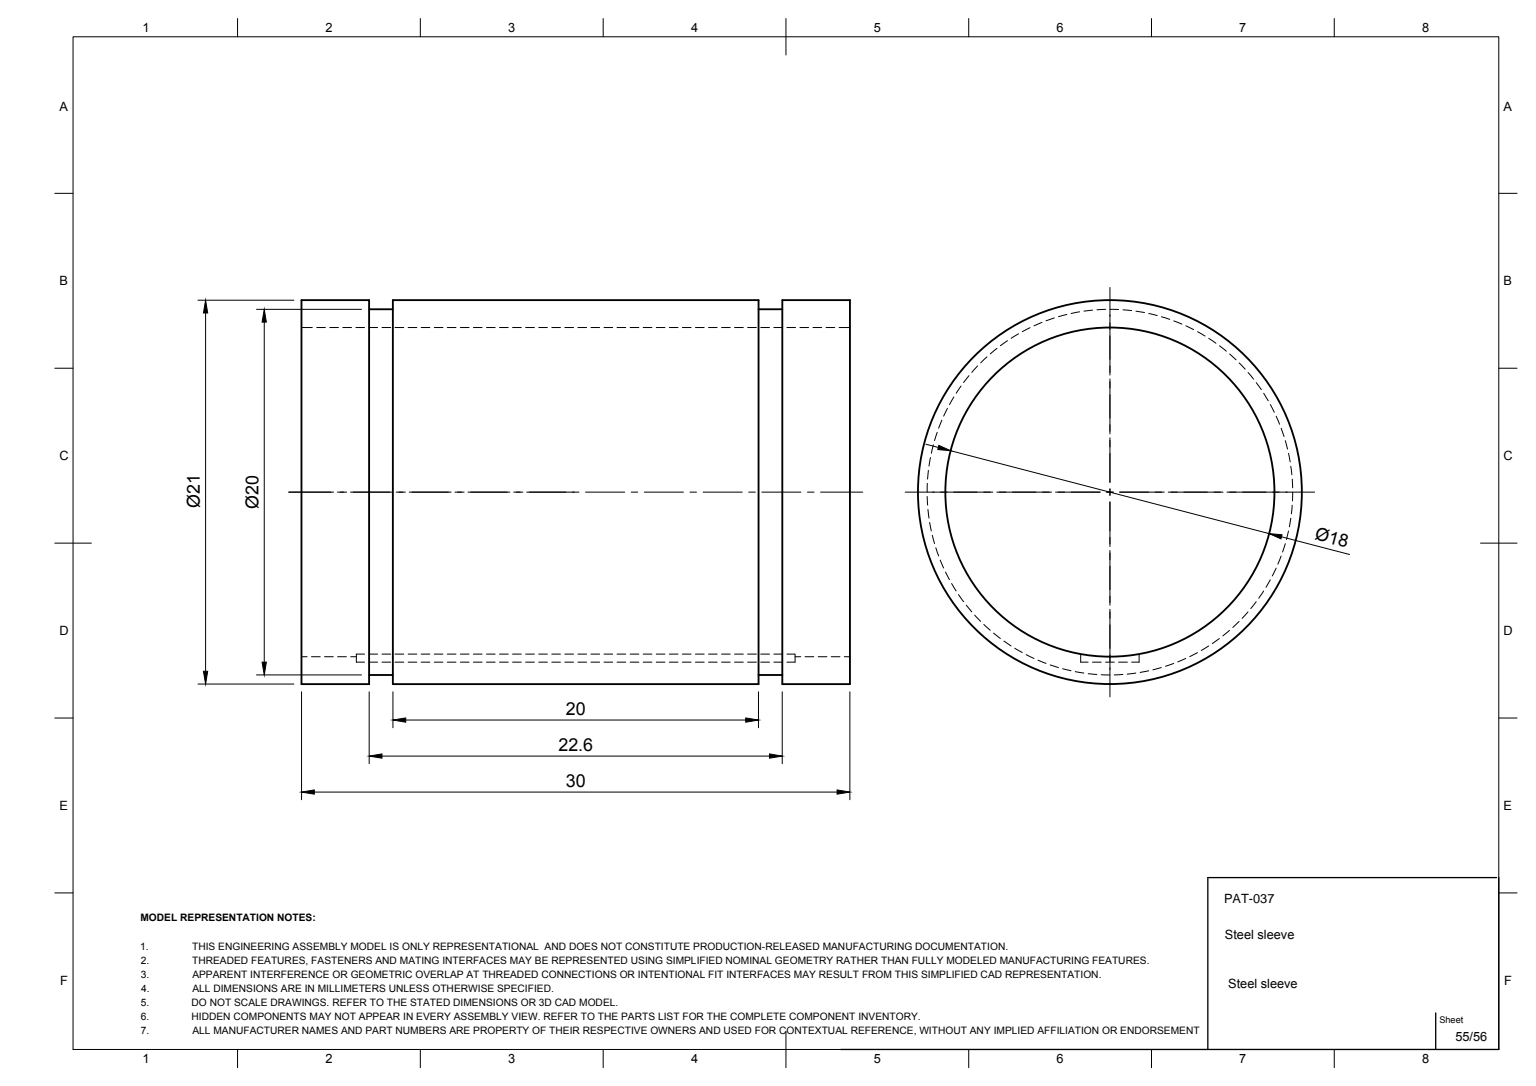
ISO-10303-21;
HEADER;
/* Generated by software containing ST-Developer
 * from STEP Tools, Inc. (www.steptools.com) 
 */

FILE_DESCRIPTION(
/* description */ ('Flywheel Crank-Slider'),
/* implementation_level */ '2;1');

FILE_NAME(
/* name */ 'Steel sleeve.step',
/* time_stamp */ '2026-10-28T03:23:13-07:00',
/* author */ (''),
/* organization */ (''),
/* preprocessor_version */ 'ST-DEVELOPER v20.2',
/* originating_system */ 'Autodesk Translation Framework v15.17.0.0',
/* authorisation */ '');

FILE_SCHEMA (('AUTOMOTIVE_DESIGN { 1 0 10303 214 3 1 1 }'));
ENDSEC;

DATA;
#10=MECHANICAL_DESIGN_GEOMETRIC_PRESENTATION_REPRESENTATION('',(#726),#17322);
#613=SHAPE_REPRESENTATION_RELATIONSHIP('SRR','None',#17615,#665);
#665=ADVANCED_BREP_SHAPE_REPRESENTATION('',(#783),#17319);
#726=STYLED_ITEM('',(#17945),#783);
#783=MANIFOLD_SOLID_BREP('Body1',#9108);
#999=FACE_BOUND('',#2569,.T.);
#1000=FACE_BOUND('',#2572,.T.);
#1001=FACE_BOUND('',#2575,.T.);
#1002=FACE_BOUND('',#2578,.T.);
#1003=FACE_BOUND('',#2581,.T.);
#1004=FACE_BOUND('',#2584,.T.);
#1005=FACE_BOUND('',#2586,.T.);
#1292=PLANE('',#10661);
#1293=PLANE('',#10663);
#1294=PLANE('',#10664);
#1295=PLANE('',#10666);
#1296=PLANE('',#10667);
#1297=PLANE('',#10668);
#1298=PLANE('',#10673);
#1299=PLANE('',#10677);
#1300=PLANE('',#10681);
#1301=PLANE('',#10685);
#1302=PLANE('',#10689);
#1814=FACE_OUTER_BOUND('',#2563,.T.);
#1815=FACE_OUTER_BOUND('',#2564,.T.);
#1816=FACE_OUTER_BOUND('',#2565,.T.);
#1817=FACE_OUTER_BOUND('',#2566,.T.);
#1818=FACE_OUTER_BOUND('',#2567,.T.);
#1819=FACE_OUTER_BOUND('',#2568,.T.);
#1820=FACE_OUTER_BOUND('',#2570,.T.);
#1821=FACE_OUTER_BOUND('',#2571,.T.);
#1822=FACE_OUTER_BOUND('',#2573,.T.);
#1823=FACE_OUTER_BOUND('',#2574,.T.);
#1824=FACE_OUTER_BOUND('',#2576,.T.);
#1825=FACE_OUTER_BOUND('',#2577,.T.);
#1826=FACE_OUTER_BOUND('',#2579,.T.);
#1827=FACE_OUTER_BOUND('',#2580,.T.);
#1828=FACE_OUTER_BOUND('',#2582,.T.);
#1829=FACE_OUTER_BOUND('',#2583,.T.);
#1830=FACE_OUTER_BOUND('',#2585,.T.);
#2563=EDGE_LOOP('',(#8174,#8175,#8176,#8177));
#2564=EDGE_LOOP('',(#8178,#8179,#8180,#8181));
#2565=EDGE_LOOP('',(#8182,#8183,#8184,#8185));
#2566=EDGE_LOOP('',(#8186,#8187,#8188,#8189));
#2567=EDGE_LOOP('',(#8190,#8191,#8192,#8193));
#2568=EDGE_LOOP('',(#8194));
#2569=EDGE_LOOP('',(#8195));
#2570=EDGE_LOOP('',(#8196,#8197,#8198,#8199));
#2571=EDGE_LOOP('',(#8200));
#2572=EDGE_LOOP('',(#8201));
#2573=EDGE_LOOP('',(#8202,#8203,#8204,#8205));
#2574=EDGE_LOOP('',(#8206));
#2575=EDGE_LOOP('',(#8207));
#2576=EDGE_LOOP('',(#8208,#8209,#8210,#8211));
#2577=EDGE_LOOP('',(#8212));
#2578=EDGE_LOOP('',(#8213));
#2579=EDGE_LOOP('',(#8214,#8215,#8216,#8217));
#2580=EDGE_LOOP('',(#8218));
#2581=EDGE_LOOP('',(#8219));
#2582=EDGE_LOOP('',(#8220,#8221,#8222,#8223));
#2583=EDGE_LOOP('',(#8224));
#2584=EDGE_LOOP('',(#8225));
#2585=EDGE_LOOP('',(#8226,#8227,#8228,#8229));
#2586=EDGE_LOOP('',(#8230,#8231,#8232,#8233));
#3178=LINE('',#16937,#3789);
#3179=LINE('',#16939,#3790);
#3180=LINE('',#16940,#3791);
#3181=LINE('',#16943,#3792);
#3182=LINE('',#16945,#3793);
#3183=LINE('',#16946,#3794);
#3184=LINE('',#16951,#3795);
#3185=LINE('',#16952,#3796);
#3186=LINE('',#16954,#3797);
#3187=LINE('',#16955,#3798);
#3188=LINE('',#16965,#3799);
#3189=LINE('',#16972,#3800);
#3190=LINE('',#16979,#3801);
#3191=LINE('',#16986,#3802);
#3192=LINE('',#16993,#3803);
#3193=LINE('',#16998,#3804);
#3789=VECTOR('',#13348,1.);
#3790=VECTOR('',#13349,1.);
#3791=VECTOR('',#13350,1.);
#3792=VECTOR('',#13353,1.);
#3793=VECTOR('',#13354,1.);
#3794=VECTOR('',#13355,1.);
#3795=VECTOR('',#13360,1.);
#3796=VECTOR('',#13361,1.);
#3797=VECTOR('',#13364,1.);
#3798=VECTOR('',#13365,1.);
#3799=VECTOR('',#13378,1.05);
#3800=VECTOR('',#13387,1.);
#3801=VECTOR('',#13396,1.05);
#3802=VECTOR('',#13405,1.);
#3803=VECTOR('',#13414,1.05);
#3804=VECTOR('',#13421,0.9);
#4248=CIRCLE('',#10662,0.9);
#4249=CIRCLE('',#10665,0.9);
#4250=CIRCLE('',#10669,1.05);
#4251=CIRCLE('',#10670,0.9);
#4252=CIRCLE('',#10672,1.05);
#4253=CIRCLE('',#10674,1.);
#4254=CIRCLE('',#10676,1.);
#4255=CIRCLE('',#10678,1.05);
#4256=CIRCLE('',#10680,1.05);
#4257=CIRCLE('',#10682,1.);
#4258=CIRCLE('',#10684,1.);
#4259=CIRCLE('',#10686,1.05);
#4260=CIRCLE('',#10688,1.05);
#4261=CIRCLE('',#10690,0.9);
#4967=VERTEX_POINT('',#16933);
#4968=VERTEX_POINT('',#16934);
#4969=VERTEX_POINT('',#16936);
#4970=VERTEX_POINT('',#16938);
#4971=VERTEX_POINT('',#16942);
#4972=VERTEX_POINT('',#16944);
#4973=VERTEX_POINT('',#16948);
#4974=VERTEX_POINT('',#16950);
#4975=VERTEX_POINT('',#16958);
#4976=VERTEX_POINT('',#16960);
#4977=VERTEX_POINT('',#16963);
#4978=VERTEX_POINT('',#16967);
#4979=VERTEX_POINT('',#16970);
#4980=VERTEX_POINT('',#16974);
#4981=VERTEX_POINT('',#16977);
#4982=VERTEX_POINT('',#16981);
#4983=VERTEX_POINT('',#16984);
#4984=VERTEX_POINT('',#16988);
#4985=VERTEX_POINT('',#16991);
#4986=VERTEX_POINT('',#16995);
#6044=EDGE_CURVE('',#4967,#4968,#4248,.T.);
#6045=EDGE_CURVE('',#4969,#4967,#3178,.T.);
#6046=EDGE_CURVE('',#4970,#4969,#3179,.T.);
#6047=EDGE_CURVE('',#4968,#4970,#3180,.T.);
#6048=EDGE_CURVE('',#4968,#4971,#3181,.T.);
#6049=EDGE_CURVE('',#4972,#4970,#3182,.T.);
#6050=EDGE_CURVE('',#4972,#4971,#3183,.T.);
#6051=EDGE_CURVE('',#4971,#4973,#4249,.T.);
#6052=EDGE_CURVE('',#4974,#4972,#3184,.T.);
#6053=EDGE_CURVE('',#4973,#4974,#3185,.T.);
#6054=EDGE_CURVE('',#4973,#4967,#3186,.T.);
#6055=EDGE_CURVE('',#4974,#4969,#3187,.T.);
#6056=EDGE_CURVE('',#4975,#4975,#4250,.T.);
#6057=EDGE_CURVE('',#4976,#4976,#4251,.T.);
#6058=EDGE_CURVE('',#4977,#4977,#4252,.T.);
#6059=EDGE_CURVE('',#4977,#4975,#3188,.T.);
#6060=EDGE_CURVE('',#4978,#4978,#4253,.T.);
#6061=EDGE_CURVE('',#4979,#4979,#4254,.T.);
#6062=EDGE_CURVE('',#4979,#4978,#3189,.T.);
#6063=EDGE_CURVE('',#4980,#4980,#4255,.T.);
#6064=EDGE_CURVE('',#4981,#4981,#4256,.T.);
#6065=EDGE_CURVE('',#4981,#4980,#3190,.T.);
#6066=EDGE_CURVE('',#4982,#4982,#4257,.T.);
#6067=EDGE_CURVE('',#4983,#4983,#4258,.T.);
#6068=EDGE_CURVE('',#4983,#4982,#3191,.T.);
#6069=EDGE_CURVE('',#4984,#4984,#4259,.T.);
#6070=EDGE_CURVE('',#4985,#4985,#4260,.T.);
#6071=EDGE_CURVE('',#4985,#4984,#3192,.T.);
#6072=EDGE_CURVE('',#4986,#4986,#4261,.T.);
#6073=EDGE_CURVE('',#4986,#4976,#3193,.T.);
#8174=ORIENTED_EDGE('',*,*,#6044,.F.);
#8175=ORIENTED_EDGE('',*,*,#6045,.F.);
#8176=ORIENTED_EDGE('',*,*,#6046,.F.);
#8177=ORIENTED_EDGE('',*,*,#6047,.F.);
#8178=ORIENTED_EDGE('',*,*,#6048,.F.);
#8179=ORIENTED_EDGE('',*,*,#6047,.T.);
#8180=ORIENTED_EDGE('',*,*,#6049,.F.);
#8181=ORIENTED_EDGE('',*,*,#6050,.T.);
#8182=ORIENTED_EDGE('',*,*,#6051,.F.);
#8183=ORIENTED_EDGE('',*,*,#6050,.F.);
#8184=ORIENTED_EDGE('',*,*,#6052,.F.);
#8185=ORIENTED_EDGE('',*,*,#6053,.F.);
#8186=ORIENTED_EDGE('',*,*,#6054,.F.);
#8187=ORIENTED_EDGE('',*,*,#6053,.T.);
#8188=ORIENTED_EDGE('',*,*,#6055,.T.);
#8189=ORIENTED_EDGE('',*,*,#6045,.T.);
#8190=ORIENTED_EDGE('',*,*,#6055,.F.);
#8191=ORIENTED_EDGE('',*,*,#6052,.T.);
#8192=ORIENTED_EDGE('',*,*,#6049,.T.);
#8193=ORIENTED_EDGE('',*,*,#6046,.T.);
#8194=ORIENTED_EDGE('',*,*,#6056,.F.);
#8195=ORIENTED_EDGE('',*,*,#6057,.T.);
#8196=ORIENTED_EDGE('',*,*,#6058,.F.);
#8197=ORIENTED_EDGE('',*,*,#6059,.T.);
#8198=ORIENTED_EDGE('',*,*,#6056,.T.);
#8199=ORIENTED_EDGE('',*,*,#6059,.F.);
#8200=ORIENTED_EDGE('',*,*,#6058,.T.);
#8201=ORIENTED_EDGE('',*,*,#6060,.F.);
#8202=ORIENTED_EDGE('',*,*,#6061,.F.);
#8203=ORIENTED_EDGE('',*,*,#6062,.T.);
#8204=ORIENTED_EDGE('',*,*,#6060,.T.);
#8205=ORIENTED_EDGE('',*,*,#6062,.F.);
#8206=ORIENTED_EDGE('',*,*,#6063,.F.);
#8207=ORIENTED_EDGE('',*,*,#6061,.T.);
#8208=ORIENTED_EDGE('',*,*,#6064,.F.);
#8209=ORIENTED_EDGE('',*,*,#6065,.T.);
#8210=ORIENTED_EDGE('',*,*,#6063,.T.);
#8211=ORIENTED_EDGE('',*,*,#6065,.F.);
#8212=ORIENTED_EDGE('',*,*,#6064,.T.);
#8213=ORIENTED_EDGE('',*,*,#6066,.F.);
#8214=ORIENTED_EDGE('',*,*,#6067,.F.);
#8215=ORIENTED_EDGE('',*,*,#6068,.T.);
#8216=ORIENTED_EDGE('',*,*,#6066,.T.);
#8217=ORIENTED_EDGE('',*,*,#6068,.F.);
#8218=ORIENTED_EDGE('',*,*,#6069,.F.);
#8219=ORIENTED_EDGE('',*,*,#6067,.T.);
#8220=ORIENTED_EDGE('',*,*,#6070,.F.);
#8221=ORIENTED_EDGE('',*,*,#6071,.T.);
#8222=ORIENTED_EDGE('',*,*,#6069,.T.);
#8223=ORIENTED_EDGE('',*,*,#6071,.F.);
#8224=ORIENTED_EDGE('',*,*,#6070,.T.);
#8225=ORIENTED_EDGE('',*,*,#6072,.F.);
#8226=ORIENTED_EDGE('',*,*,#6072,.T.);
#8227=ORIENTED_EDGE('',*,*,#6073,.T.);
#8228=ORIENTED_EDGE('',*,*,#6057,.F.);
#8229=ORIENTED_EDGE('',*,*,#6073,.F.);
#8230=ORIENTED_EDGE('',*,*,#6051,.T.);
#8231=ORIENTED_EDGE('',*,*,#6054,.T.);
#8232=ORIENTED_EDGE('',*,*,#6044,.T.);
#8233=ORIENTED_EDGE('',*,*,#6048,.T.);
#8501=CYLINDRICAL_SURFACE('',#10671,1.05);
#8502=CYLINDRICAL_SURFACE('',#10675,1.);
#8503=CYLINDRICAL_SURFACE('',#10679,1.05);
#8504=CYLINDRICAL_SURFACE('',#10683,1.);
#8505=CYLINDRICAL_SURFACE('',#10687,1.05);
#8506=CYLINDRICAL_SURFACE('',#10691,0.9);
#9005=ADVANCED_FACE('',(#1814),#1292,.F.);
#9006=ADVANCED_FACE('',(#1815),#1293,.F.);
#9007=ADVANCED_FACE('',(#1816),#1294,.F.);
#9008=ADVANCED_FACE('',(#1817),#1295,.F.);
#9009=ADVANCED_FACE('',(#1818),#1296,.F.);
#9010=ADVANCED_FACE('',(#1819,#999),#1297,.T.);
#9011=ADVANCED_FACE('',(#1820),#8501,.T.);
#9012=ADVANCED_FACE('',(#1821,#1000),#1298,.T.);
#9013=ADVANCED_FACE('',(#1822),#8502,.T.);
#9014=ADVANCED_FACE('',(#1823,#1001),#1299,.T.);
#9015=ADVANCED_FACE('',(#1824),#8503,.T.);
#9016=ADVANCED_FACE('',(#1825,#1002),#1300,.T.);
#9017=ADVANCED_FACE('',(#1826),#8504,.T.);
#9018=ADVANCED_FACE('',(#1827,#1003),#1301,.T.);
#9019=ADVANCED_FACE('',(#1828),#8505,.T.);
#9020=ADVANCED_FACE('',(#1829,#1004),#1302,.T.);
#9021=ADVANCED_FACE('',(#1830,#1005),#8506,.F.);
#9108=CLOSED_SHELL('',(#9005,#9006,#9007,#9008,#9009,#9010,#9011,#9012,
#9013,#9014,#9015,#9016,#9017,#9018,#9019,#9020,#9021));
#10660=AXIS2_PLACEMENT_3D('',#16931,#13342,#13343);
#10661=AXIS2_PLACEMENT_3D('',#16932,#13344,#13345);
#10662=AXIS2_PLACEMENT_3D('',#16935,#13346,#13347);
#10663=AXIS2_PLACEMENT_3D('',#16941,#13351,#13352);
#10664=AXIS2_PLACEMENT_3D('',#16947,#13356,#13357);
#10665=AXIS2_PLACEMENT_3D('',#16949,#13358,#13359);
#10666=AXIS2_PLACEMENT_3D('',#16953,#13362,#13363);
#10667=AXIS2_PLACEMENT_3D('',#16956,#13366,#13367);
#10668=AXIS2_PLACEMENT_3D('',#16957,#13368,#13369);
#10669=AXIS2_PLACEMENT_3D('',#16959,#13370,#13371);
#10670=AXIS2_PLACEMENT_3D('',#16961,#13372,#13373);
#10671=AXIS2_PLACEMENT_3D('',#16962,#13374,#13375);
#10672=AXIS2_PLACEMENT_3D('',#16964,#13376,#13377);
#10673=AXIS2_PLACEMENT_3D('',#16966,#13379,#13380);
#10674=AXIS2_PLACEMENT_3D('',#16968,#13381,#13382);
#10675=AXIS2_PLACEMENT_3D('',#16969,#13383,#13384);
#10676=AXIS2_PLACEMENT_3D('',#16971,#13385,#13386);
#10677=AXIS2_PLACEMENT_3D('',#16973,#13388,#13389);
#10678=AXIS2_PLACEMENT_3D('',#16975,#13390,#13391);
#10679=AXIS2_PLACEMENT_3D('',#16976,#13392,#13393);
#10680=AXIS2_PLACEMENT_3D('',#16978,#13394,#13395);
#10681=AXIS2_PLACEMENT_3D('',#16980,#13397,#13398);
#10682=AXIS2_PLACEMENT_3D('',#16982,#13399,#13400);
#10683=AXIS2_PLACEMENT_3D('',#16983,#13401,#13402);
#10684=AXIS2_PLACEMENT_3D('',#16985,#13403,#13404);
#10685=AXIS2_PLACEMENT_3D('',#16987,#13406,#13407);
#10686=AXIS2_PLACEMENT_3D('',#16989,#13408,#13409);
#10687=AXIS2_PLACEMENT_3D('',#16990,#13410,#13411);
#10688=AXIS2_PLACEMENT_3D('',#16992,#13412,#13413);
#10689=AXIS2_PLACEMENT_3D('',#16994,#13415,#13416);
#10690=AXIS2_PLACEMENT_3D('',#16996,#13417,#13418);
#10691=AXIS2_PLACEMENT_3D('',#16997,#13419,#13420);
#13342=DIRECTION('axis',(0.,0.,1.));
#13343=DIRECTION('refdir',(1.,0.,0.));
#13344=DIRECTION('center_axis',(0.,1.,0.));
#13345=DIRECTION('ref_axis',(0.,0.,1.));
#13346=DIRECTION('center_axis',(0.,-1.,0.));
#13347=DIRECTION('ref_axis',(1.,0.,0.));
#13348=DIRECTION('',(-1.,0.,0.));
#13349=DIRECTION('',(0.,0.,-1.));
#13350=DIRECTION('',(1.,0.,0.));
#13351=DIRECTION('center_axis',(0.,0.,1.));
#13352=DIRECTION('ref_axis',(1.,0.,0.));
#13353=DIRECTION('',(0.,-1.,0.));
#13354=DIRECTION('',(0.,1.,0.));
#13355=DIRECTION('',(-1.,0.,0.));
#13356=DIRECTION('center_axis',(0.,-1.,0.));
#13357=DIRECTION('ref_axis',(0.,0.,-1.));
#13358=DIRECTION('center_axis',(0.,1.,0.));
#13359=DIRECTION('ref_axis',(1.,0.,0.));
#13360=DIRECTION('',(0.,0.,1.));
#13361=DIRECTION('',(1.,0.,0.));
#13362=DIRECTION('center_axis',(0.,0.,-1.));
#13363=DIRECTION('ref_axis',(-1.,0.,0.));
#13364=DIRECTION('',(0.,1.,0.));
#13365=DIRECTION('',(0.,1.,0.));
#13366=DIRECTION('center_axis',(1.,0.,0.));
#13367=DIRECTION('ref_axis',(0.,0.,-1.));
#13368=DIRECTION('center_axis',(0.,1.,0.));
#13369=DIRECTION('ref_axis',(0.,0.,1.));
#13370=DIRECTION('center_axis',(0.,-1.,0.));
#13371=DIRECTION('ref_axis',(1.,0.,0.));
#13372=DIRECTION('center_axis',(0.,-1.,0.));
#13373=DIRECTION('ref_axis',(1.,0.,0.));
#13374=DIRECTION('center_axis',(0.,-1.,0.));
#13375=DIRECTION('ref_axis',(1.,0.,0.));
#13376=DIRECTION('center_axis',(0.,-1.,0.));
#13377=DIRECTION('ref_axis',(1.,0.,0.));
#13378=DIRECTION('',(0.,1.,0.));
#13379=DIRECTION('center_axis',(0.,-1.,0.));
#13380=DIRECTION('ref_axis',(0.,0.,-1.));
#13381=DIRECTION('center_axis',(0.,-1.,0.));
#13382=DIRECTION('ref_axis',(1.,0.,0.));
#13383=DIRECTION('center_axis',(0.,-1.,0.));
#13384=DIRECTION('ref_axis',(1.,0.,0.));
#13385=DIRECTION('center_axis',(0.,-1.,0.));
#13386=DIRECTION('ref_axis',(1.,0.,0.));
#13387=DIRECTION('',(0.,1.,0.));
#13388=DIRECTION('center_axis',(0.,1.,0.));
#13389=DIRECTION('ref_axis',(0.,0.,1.));
#13390=DIRECTION('center_axis',(0.,-1.,0.));
#13391=DIRECTION('ref_axis',(1.,0.,0.));
#13392=DIRECTION('center_axis',(0.,-1.,0.));
#13393=DIRECTION('ref_axis',(1.,0.,0.));
#13394=DIRECTION('center_axis',(0.,-1.,0.));
#13395=DIRECTION('ref_axis',(1.,0.,0.));
#13396=DIRECTION('',(0.,1.,0.));
#13397=DIRECTION('center_axis',(0.,-1.,0.));
#13398=DIRECTION('ref_axis',(0.,0.,-1.));
#13399=DIRECTION('center_axis',(0.,-1.,0.));
#13400=DIRECTION('ref_axis',(1.,0.,0.));
#13401=DIRECTION('center_axis',(0.,-1.,0.));
#13402=DIRECTION('ref_axis',(1.,0.,0.));
#13403=DIRECTION('center_axis',(0.,-1.,0.));
#13404=DIRECTION('ref_axis',(1.,0.,0.));
#13405=DIRECTION('',(0.,1.,0.));
#13406=DIRECTION('center_axis',(0.,1.,0.));
#13407=DIRECTION('ref_axis',(0.,0.,1.));
#13408=DIRECTION('center_axis',(0.,-1.,0.));
#13409=DIRECTION('ref_axis',(1.,0.,0.));
#13410=DIRECTION('center_axis',(0.,-1.,0.));
#13411=DIRECTION('ref_axis',(1.,0.,0.));
#13412=DIRECTION('center_axis',(0.,-1.,0.));
#13413=DIRECTION('ref_axis',(1.,0.,0.));
#13414=DIRECTION('',(0.,1.,0.));
#13415=DIRECTION('center_axis',(0.,-1.,0.));
#13416=DIRECTION('ref_axis',(0.,0.,-1.));
#13417=DIRECTION('center_axis',(0.,-1.,0.));
#13418=DIRECTION('ref_axis',(1.,0.,0.));
#13419=DIRECTION('center_axis',(0.,-1.,0.));
#13420=DIRECTION('ref_axis',(1.,0.,0.));
#13421=DIRECTION('',(0.,1.,0.));
#16931=CARTESIAN_POINT('',(0.,0.,0.));
#16932=CARTESIAN_POINT('Origin',(0.75,1.2,0.));
#16933=CARTESIAN_POINT('',(0.885663593019381,1.2,-0.16));
#16934=CARTESIAN_POINT('',(0.885663593019381,1.2,0.16));
#16935=CARTESIAN_POINT('Origin',(0.,1.2,0.));
#16936=CARTESIAN_POINT('',(0.93,1.2,-0.16));
#16937=CARTESIAN_POINT('',(0.93,1.2,-0.16));
#16938=CARTESIAN_POINT('',(0.93,1.2,0.16));
#16939=CARTESIAN_POINT('',(0.93,1.2,0.16));
#16940=CARTESIAN_POINT('',(0.57,1.2,0.16));
#16941=CARTESIAN_POINT('Origin',(0.57,0.,0.16));
#16942=CARTESIAN_POINT('',(0.885663593019381,-1.2,0.16));
#16943=CARTESIAN_POINT('',(0.885663593019381,0.,0.16));
#16944=CARTESIAN_POINT('',(0.93,-1.2,0.16));
#16945=CARTESIAN_POINT('',(0.93,0.,0.16));
#16946=CARTESIAN_POINT('',(0.57,-1.2,0.16));
#16947=CARTESIAN_POINT('Origin',(0.75,-1.2,0.));
#16948=CARTESIAN_POINT('',(0.885663593019381,-1.2,-0.16));
#16949=CARTESIAN_POINT('Origin',(0.,-1.2,0.));
#16950=CARTESIAN_POINT('',(0.93,-1.2,-0.16));
#16951=CARTESIAN_POINT('',(0.93,-1.2,0.16));
#16952=CARTESIAN_POINT('',(0.93,-1.2,-0.16));
#16953=CARTESIAN_POINT('Origin',(0.93,0.,-0.16));
#16954=CARTESIAN_POINT('',(0.885663593019381,0.,-0.16));
#16955=CARTESIAN_POINT('',(0.93,0.,-0.16));
#16956=CARTESIAN_POINT('Origin',(0.93,0.,0.16));
#16957=CARTESIAN_POINT('Origin',(1.05,1.5,0.));
#16958=CARTESIAN_POINT('',(-1.05,1.5,-1.28587913910472E-16));
#16959=CARTESIAN_POINT('Origin',(0.,1.5,0.));
#16960=CARTESIAN_POINT('',(-0.9,1.5,-1.10218211923262E-16));
#16961=CARTESIAN_POINT('Origin',(0.,1.5,0.));
#16962=CARTESIAN_POINT('Origin',(0.,1.315,0.));
#16963=CARTESIAN_POINT('',(-1.05,1.13,-1.28587913910472E-16));
#16964=CARTESIAN_POINT('Origin',(0.,1.13,0.));
#16965=CARTESIAN_POINT('',(-1.05,1.315,-1.28587913910472E-16));
#16966=CARTESIAN_POINT('Origin',(1.,1.13,0.));
#16967=CARTESIAN_POINT('',(-1.,1.13,-1.22464679914735E-16));
#16968=CARTESIAN_POINT('Origin',(0.,1.13,0.));
#16969=CARTESIAN_POINT('Origin',(0.,1.065,0.));
#16970=CARTESIAN_POINT('',(-1.,1.,-1.22464679914735E-16));
#16971=CARTESIAN_POINT('Origin',(0.,1.,0.));
#16972=CARTESIAN_POINT('',(-1.,1.065,-1.22464679914735E-16));
#16973=CARTESIAN_POINT('Origin',(1.05,1.,0.));
#16974=CARTESIAN_POINT('',(-1.05,1.,-1.28587913910472E-16));
#16975=CARTESIAN_POINT('Origin',(0.,1.,0.));
#16976=CARTESIAN_POINT('Origin',(0.,0.,0.));
#16977=CARTESIAN_POINT('',(-1.05,-1.,-1.28587913910472E-16));
#16978=CARTESIAN_POINT('Origin',(0.,-1.,0.));
#16979=CARTESIAN_POINT('',(-1.05,0.,-1.28587913910472E-16));
#16980=CARTESIAN_POINT('Origin',(1.,-1.,0.));
#16981=CARTESIAN_POINT('',(-1.,-1.,-1.22464679914735E-16));
#16982=CARTESIAN_POINT('Origin',(0.,-1.,0.));
#16983=CARTESIAN_POINT('Origin',(0.,-1.065,0.));
#16984=CARTESIAN_POINT('',(-1.,-1.13,-1.22464679914735E-16));
#16985=CARTESIAN_POINT('Origin',(0.,-1.13,0.));
#16986=CARTESIAN_POINT('',(-1.,-1.065,-1.22464679914735E-16));
#16987=CARTESIAN_POINT('Origin',(1.05,-1.13,0.));
#16988=CARTESIAN_POINT('',(-1.05,-1.13,-1.28587913910472E-16));
#16989=CARTESIAN_POINT('Origin',(0.,-1.13,0.));
#16990=CARTESIAN_POINT('Origin',(0.,-1.315,0.));
#16991=CARTESIAN_POINT('',(-1.05,-1.5,-1.28587913910472E-16));
#16992=CARTESIAN_POINT('Origin',(0.,-1.5,0.));
#16993=CARTESIAN_POINT('',(-1.05,-1.315,-1.28587913910472E-16));
#16994=CARTESIAN_POINT('Origin',(0.9,-1.5,0.));
#16995=CARTESIAN_POINT('',(-0.9,-1.5,-1.10218211923262E-16));
#16996=CARTESIAN_POINT('Origin',(0.,-1.5,0.));
#16997=CARTESIAN_POINT('Origin',(0.,0.,0.));
#16998=CARTESIAN_POINT('',(-0.9,0.,-1.10218211923262E-16));
#17258=UNCERTAINTY_MEASURE_WITH_UNIT(LENGTH_MEASURE(0.001),#17323,
'DISTANCE_ACCURACY_VALUE',
'Maximum model space distance between geometric entities at asserted c
onnectivities');
#17261=UNCERTAINTY_MEASURE_WITH_UNIT(LENGTH_MEASURE(0.001),#17323,
'DISTANCE_ACCURACY_VALUE',
'Maximum model space distance between geometric entities at asserted c
onnectivities');
#17319=(
GEOMETRIC_REPRESENTATION_CONTEXT(3)
GLOBAL_UNCERTAINTY_ASSIGNED_CONTEXT((#17258))
GLOBAL_UNIT_ASSIGNED_CONTEXT((#17323,#17325,#17326))
REPRESENTATION_CONTEXT('','3D')
);
#17322=(
GEOMETRIC_REPRESENTATION_CONTEXT(3)
GLOBAL_UNCERTAINTY_ASSIGNED_CONTEXT((#17261))
GLOBAL_UNIT_ASSIGNED_CONTEXT((#17323,#17325,#17326))
REPRESENTATION_CONTEXT('','3D')
);
#17323=(
LENGTH_UNIT()
NAMED_UNIT(*)
SI_UNIT(.CENTI.,.METRE.)
);
#17325=(
NAMED_UNIT(*)
PLANE_ANGLE_UNIT()
SI_UNIT($,.RADIAN.)
);
#17326=(
NAMED_UNIT(*)
SI_UNIT($,.STERADIAN.)
SOLID_ANGLE_UNIT()
);
#17384=SHAPE_DEFINITION_REPRESENTATION(#17458,#17615);
#17458=PRODUCT_DEFINITION_SHAPE('',$,#17676);
#17615=SHAPE_REPRESENTATION('',(#10660),#17319);
#17618=PRODUCT_DEFINITION_CONTEXT('part definition',#17800,'design');
#17676=PRODUCT_DEFINITION('Steel sleeve','Steel sleeve',#17736,#17618);
#17736=PRODUCT_DEFINITION_FORMATION('',$,#17859);
#17800=APPLICATION_CONTEXT(
'Core Data for Automotive Mechanical Design Process');
#17801=PRODUCT_CONTEXT('part definition',#17800,'mechanical');
#17859=PRODUCT('Steel sleeve','Steel sleeve','Steel sleeve',(#17801));
#17939=COLOUR_RGB('Off White',0.89,0.88,0.83);
#17940=FILL_AREA_STYLE_COLOUR('',#17939);
#17941=FILL_AREA_STYLE('',(#17940));
#17942=SURFACE_STYLE_FILL_AREA(#17941);
#17943=SURFACE_SIDE_STYLE('',(#17942));
#17944=SURFACE_STYLE_USAGE(.BOTH.,#17943);
#17945=PRESENTATION_STYLE_ASSIGNMENT((#17944));
ENDSEC;
END-ISO-10303-21;
